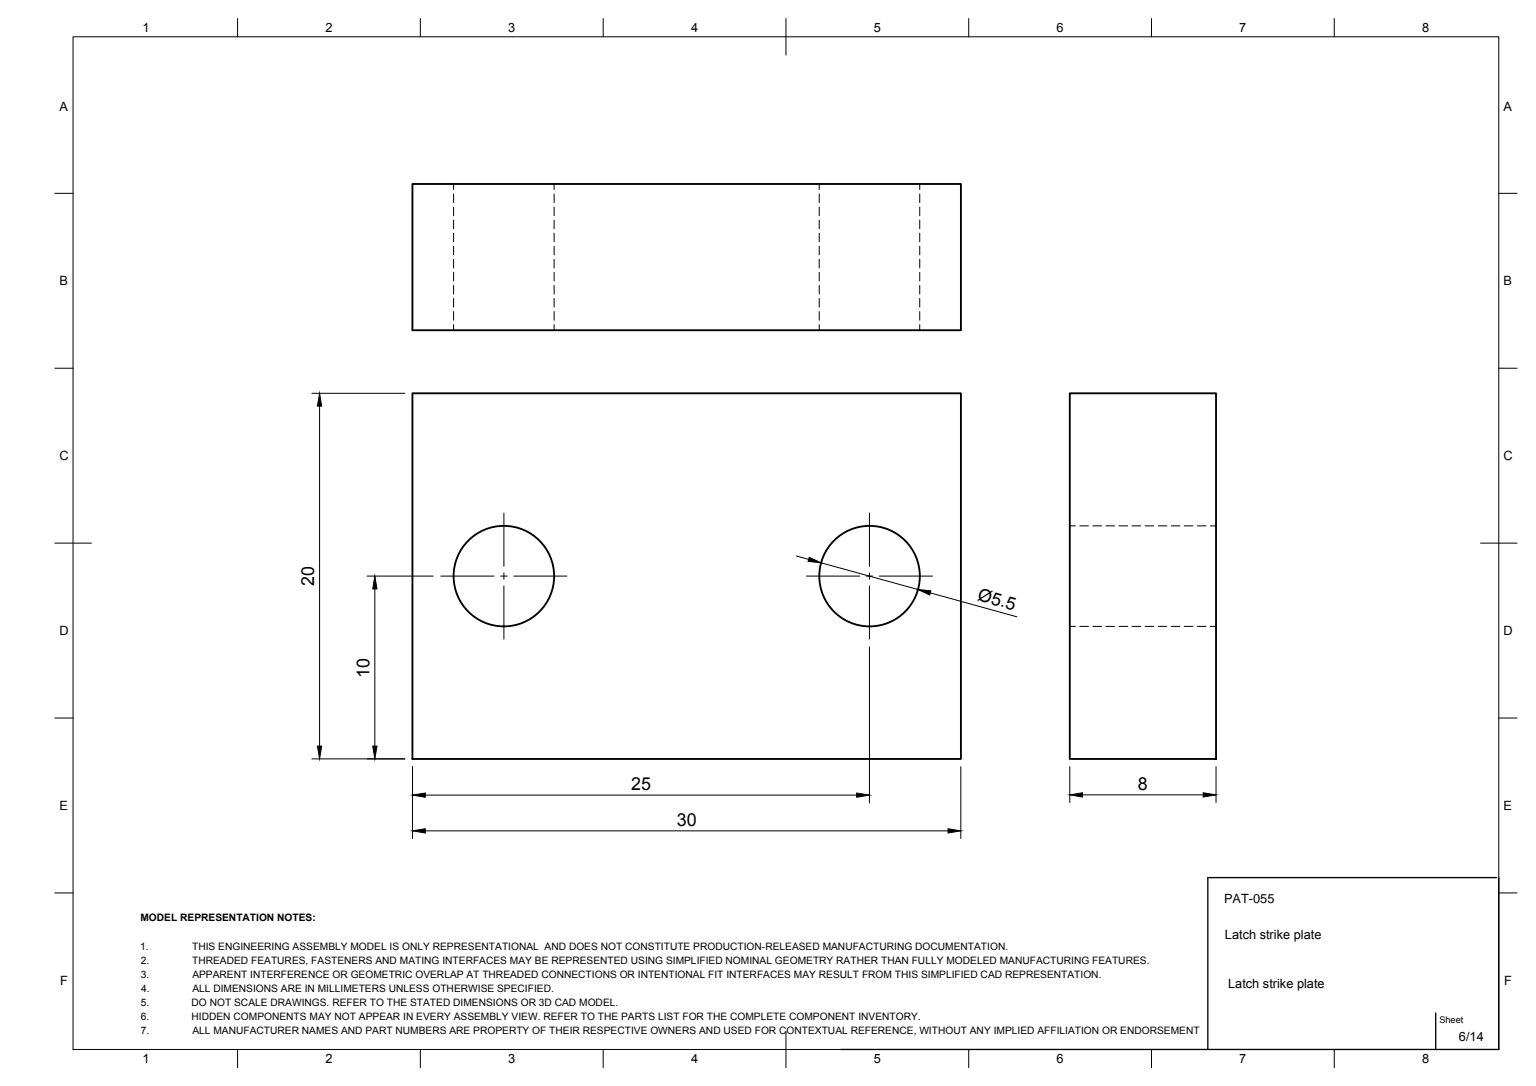
ISO-10303-21;
HEADER;
/* Generated by software containing ST-Developer
 * from STEP Tools, Inc. (www.steptools.com) 
 */

FILE_DESCRIPTION(
/* description */ ('Hinged panel with latch'),
/* implementation_level */ '2;1');

FILE_NAME(
/* name */ 'Latch strike plate.step',
/* time_stamp */ '2026-10-27T20:36:01-07:00',
/* author */ (''),
/* organization */ (''),
/* preprocessor_version */ 'ST-DEVELOPER v20.2',
/* originating_system */ 'Autodesk Translation Framework v15.17.0.0',
/* authorisation */ '');

FILE_SCHEMA (('AUTOMOTIVE_DESIGN { 1 0 10303 214 3 1 1 }'));
ENDSEC;

DATA;
#10=MECHANICAL_DESIGN_GEOMETRIC_PRESENTATION_REPRESENTATION('',(#296),#6743);
#264=SHAPE_REPRESENTATION_RELATIONSHIP('SRR','None',#6839,#280);
#280=ADVANCED_BREP_SHAPE_REPRESENTATION('',(#312),#6725);
#296=STYLED_ITEM('',(#6989),#312);
#312=MANIFOLD_SOLID_BREP('Body1',#3798);
#325=FACE_BOUND('',#732,.T.);
#326=FACE_BOUND('',#733,.T.);
#327=FACE_BOUND('',#736,.T.);
#328=FACE_BOUND('',#737,.T.);
#372=PLANE('',#4003);
#373=PLANE('',#4004);
#374=PLANE('',#4005);
#375=PLANE('',#4006);
#376=PLANE('',#4007);
#377=PLANE('',#4008);
#523=FACE_OUTER_BOUND('',#729,.T.);
#524=FACE_OUTER_BOUND('',#730,.T.);
#525=FACE_OUTER_BOUND('',#731,.T.);
#526=FACE_OUTER_BOUND('',#734,.T.);
#527=FACE_OUTER_BOUND('',#735,.T.);
#528=FACE_OUTER_BOUND('',#738,.T.);
#529=FACE_OUTER_BOUND('',#739,.T.);
#530=FACE_OUTER_BOUND('',#740,.T.);
#729=EDGE_LOOP('',(#2590,#2591,#2592,#2593));
#730=EDGE_LOOP('',(#2594,#2595,#2596,#2597));
#731=EDGE_LOOP('',(#2598,#2599,#2600,#2601));
#732=EDGE_LOOP('',(#2602));
#733=EDGE_LOOP('',(#2603));
#734=EDGE_LOOP('',(#2604,#2605,#2606,#2607));
#735=EDGE_LOOP('',(#2608,#2609,#2610,#2611));
#736=EDGE_LOOP('',(#2612));
#737=EDGE_LOOP('',(#2613));
#738=EDGE_LOOP('',(#2614,#2615,#2616,#2617));
#739=EDGE_LOOP('',(#2618,#2619,#2620,#2621));
#740=EDGE_LOOP('',(#2622,#2623,#2624,#2625));
#982=LINE('',#5469,#1340);
#983=LINE('',#5475,#1341);
#984=LINE('',#5480,#1342);
#985=LINE('',#5482,#1343);
#986=LINE('',#5484,#1344);
#987=LINE('',#5485,#1345);
#988=LINE('',#5488,#1346);
#989=LINE('',#5490,#1347);
#990=LINE('',#5491,#1348);
#991=LINE('',#5494,#1349);
#992=LINE('',#5496,#1350);
#993=LINE('',#5497,#1351);
#994=LINE('',#5499,#1352);
#995=LINE('',#5500,#1353);
#1340=VECTOR('',#4374,0.274999999999999);
#1341=VECTOR('',#4381,0.274999999999999);
#1342=VECTOR('',#4386,1.);
#1343=VECTOR('',#4387,1.);
#1344=VECTOR('',#4388,1.);
#1345=VECTOR('',#4389,1.);
#1346=VECTOR('',#4392,1.);
#1347=VECTOR('',#4393,1.);
#1348=VECTOR('',#4394,1.);
#1349=VECTOR('',#4397,1.);
#1350=VECTOR('',#4398,1.);
#1351=VECTOR('',#4399,1.);
#1352=VECTOR('',#4402,1.);
#1353=VECTOR('',#4403,1.);
#1698=CIRCLE('',#3998,0.274999999999999);
#1699=CIRCLE('',#3999,0.274999999999999);
#1700=CIRCLE('',#4001,0.274999999999999);
#1701=CIRCLE('',#4002,0.274999999999999);
#1791=VERTEX_POINT('',#5466);
#1792=VERTEX_POINT('',#5468);
#1793=VERTEX_POINT('',#5472);
#1794=VERTEX_POINT('',#5474);
#1795=VERTEX_POINT('',#5478);
#1796=VERTEX_POINT('',#5479);
#1797=VERTEX_POINT('',#5481);
#1798=VERTEX_POINT('',#5483);
#1799=VERTEX_POINT('',#5487);
#1800=VERTEX_POINT('',#5489);
#1801=VERTEX_POINT('',#5493);
#1802=VERTEX_POINT('',#5495);
#2107=EDGE_CURVE('',#1791,#1791,#1698,.T.);
#2108=EDGE_CURVE('',#1791,#1792,#982,.T.);
#2109=EDGE_CURVE('',#1792,#1792,#1699,.T.);
#2110=EDGE_CURVE('',#1793,#1793,#1700,.T.);
#2111=EDGE_CURVE('',#1793,#1794,#983,.T.);
#2112=EDGE_CURVE('',#1794,#1794,#1701,.T.);
#2113=EDGE_CURVE('',#1795,#1796,#984,.T.);
#2114=EDGE_CURVE('',#1796,#1797,#985,.T.);
#2115=EDGE_CURVE('',#1798,#1797,#986,.T.);
#2116=EDGE_CURVE('',#1795,#1798,#987,.T.);
#2117=EDGE_CURVE('',#1799,#1795,#988,.T.);
#2118=EDGE_CURVE('',#1800,#1798,#989,.T.);
#2119=EDGE_CURVE('',#1799,#1800,#990,.T.);
#2120=EDGE_CURVE('',#1801,#1799,#991,.T.);
#2121=EDGE_CURVE('',#1802,#1800,#992,.T.);
#2122=EDGE_CURVE('',#1801,#1802,#993,.T.);
#2123=EDGE_CURVE('',#1796,#1801,#994,.T.);
#2124=EDGE_CURVE('',#1797,#1802,#995,.T.);
#2590=ORIENTED_EDGE('',*,*,#2107,.F.);
#2591=ORIENTED_EDGE('',*,*,#2108,.T.);
#2592=ORIENTED_EDGE('',*,*,#2109,.F.);
#2593=ORIENTED_EDGE('',*,*,#2108,.F.);
#2594=ORIENTED_EDGE('',*,*,#2110,.F.);
#2595=ORIENTED_EDGE('',*,*,#2111,.T.);
#2596=ORIENTED_EDGE('',*,*,#2112,.F.);
#2597=ORIENTED_EDGE('',*,*,#2111,.F.);
#2598=ORIENTED_EDGE('',*,*,#2113,.T.);
#2599=ORIENTED_EDGE('',*,*,#2114,.T.);
#2600=ORIENTED_EDGE('',*,*,#2115,.F.);
#2601=ORIENTED_EDGE('',*,*,#2116,.F.);
#2602=ORIENTED_EDGE('',*,*,#2109,.T.);
#2603=ORIENTED_EDGE('',*,*,#2112,.T.);
#2604=ORIENTED_EDGE('',*,*,#2117,.T.);
#2605=ORIENTED_EDGE('',*,*,#2116,.T.);
#2606=ORIENTED_EDGE('',*,*,#2118,.F.);
#2607=ORIENTED_EDGE('',*,*,#2119,.F.);
#2608=ORIENTED_EDGE('',*,*,#2120,.T.);
#2609=ORIENTED_EDGE('',*,*,#2119,.T.);
#2610=ORIENTED_EDGE('',*,*,#2121,.F.);
#2611=ORIENTED_EDGE('',*,*,#2122,.F.);
#2612=ORIENTED_EDGE('',*,*,#2107,.T.);
#2613=ORIENTED_EDGE('',*,*,#2110,.T.);
#2614=ORIENTED_EDGE('',*,*,#2123,.T.);
#2615=ORIENTED_EDGE('',*,*,#2122,.T.);
#2616=ORIENTED_EDGE('',*,*,#2124,.F.);
#2617=ORIENTED_EDGE('',*,*,#2114,.F.);
#2618=ORIENTED_EDGE('',*,*,#2124,.T.);
#2619=ORIENTED_EDGE('',*,*,#2121,.T.);
#2620=ORIENTED_EDGE('',*,*,#2118,.T.);
#2621=ORIENTED_EDGE('',*,*,#2115,.T.);
#2622=ORIENTED_EDGE('',*,*,#2123,.F.);
#2623=ORIENTED_EDGE('',*,*,#2113,.F.);
#2624=ORIENTED_EDGE('',*,*,#2117,.F.);
#2625=ORIENTED_EDGE('',*,*,#2120,.F.);
#3556=CYLINDRICAL_SURFACE('',#3997,0.274999999999999);
#3557=CYLINDRICAL_SURFACE('',#4000,0.274999999999999);
#3592=ADVANCED_FACE('',(#523),#3556,.F.);
#3593=ADVANCED_FACE('',(#524),#3557,.F.);
#3594=ADVANCED_FACE('',(#525,#325,#326),#372,.T.);
#3595=ADVANCED_FACE('',(#526),#373,.T.);
#3596=ADVANCED_FACE('',(#527,#327,#328),#374,.T.);
#3597=ADVANCED_FACE('',(#528),#375,.T.);
#3598=ADVANCED_FACE('',(#529),#376,.T.);
#3599=ADVANCED_FACE('',(#530),#377,.F.);
#3798=CLOSED_SHELL('',(#3592,#3593,#3594,#3595,#3596,#3597,#3598,#3599));
#3996=AXIS2_PLACEMENT_3D('',#5464,#4368,#4369);
#3997=AXIS2_PLACEMENT_3D('',#5465,#4370,#4371);
#3998=AXIS2_PLACEMENT_3D('',#5467,#4372,#4373);
#3999=AXIS2_PLACEMENT_3D('',#5470,#4375,#4376);
#4000=AXIS2_PLACEMENT_3D('',#5471,#4377,#4378);
#4001=AXIS2_PLACEMENT_3D('',#5473,#4379,#4380);
#4002=AXIS2_PLACEMENT_3D('',#5476,#4382,#4383);
#4003=AXIS2_PLACEMENT_3D('',#5477,#4384,#4385);
#4004=AXIS2_PLACEMENT_3D('',#5486,#4390,#4391);
#4005=AXIS2_PLACEMENT_3D('',#5492,#4395,#4396);
#4006=AXIS2_PLACEMENT_3D('',#5498,#4400,#4401);
#4007=AXIS2_PLACEMENT_3D('',#5501,#4404,#4405);
#4008=AXIS2_PLACEMENT_3D('',#5502,#4406,#4407);
#4368=DIRECTION('axis',(0.,0.,1.));
#4369=DIRECTION('refdir',(1.,0.,0.));
#4370=DIRECTION('center_axis',(0.,1.,0.));
#4371=DIRECTION('ref_axis',(1.,0.,0.));
#4372=DIRECTION('center_axis',(0.,1.,0.));
#4373=DIRECTION('ref_axis',(1.,0.,0.));
#4374=DIRECTION('',(0.,1.,0.));
#4375=DIRECTION('center_axis',(0.,-1.,0.));
#4376=DIRECTION('ref_axis',(1.,0.,0.));
#4377=DIRECTION('center_axis',(0.,1.,0.));
#4378=DIRECTION('ref_axis',(1.,0.,0.));
#4379=DIRECTION('center_axis',(0.,1.,0.));
#4380=DIRECTION('ref_axis',(1.,0.,0.));
#4381=DIRECTION('',(0.,1.,0.));
#4382=DIRECTION('center_axis',(0.,-1.,0.));
#4383=DIRECTION('ref_axis',(1.,0.,0.));
#4384=DIRECTION('center_axis',(0.,1.,0.));
#4385=DIRECTION('ref_axis',(-1.,0.,0.));
#4386=DIRECTION('',(-1.,0.,0.));
#4387=DIRECTION('',(0.,0.,1.));
#4388=DIRECTION('',(-1.,0.,0.));
#4389=DIRECTION('',(0.,0.,1.));
#4390=DIRECTION('center_axis',(1.,0.,0.));
#4391=DIRECTION('ref_axis',(0.,1.,0.));
#4392=DIRECTION('',(0.,1.,0.));
#4393=DIRECTION('',(0.,1.,0.));
#4394=DIRECTION('',(0.,0.,1.));
#4395=DIRECTION('center_axis',(0.,-1.,0.));
#4396=DIRECTION('ref_axis',(1.,0.,0.));
#4397=DIRECTION('',(1.,0.,0.));
#4398=DIRECTION('',(1.,0.,0.));
#4399=DIRECTION('',(0.,0.,1.));
#4400=DIRECTION('center_axis',(-1.,0.,0.));
#4401=DIRECTION('ref_axis',(0.,-1.,0.));
#4402=DIRECTION('',(0.,-1.,0.));
#4403=DIRECTION('',(0.,-1.,0.));
#4404=DIRECTION('center_axis',(0.,0.,1.));
#4405=DIRECTION('ref_axis',(1.,0.,0.));
#4406=DIRECTION('center_axis',(0.,0.,1.));
#4407=DIRECTION('ref_axis',(1.,0.,0.));
#5464=CARTESIAN_POINT('',(0.,0.,0.));
#5465=CARTESIAN_POINT('Origin',(22.,-1.9,15.));
#5466=CARTESIAN_POINT('',(21.725,-1.8,15.));
#5467=CARTESIAN_POINT('Origin',(22.,-1.8,15.));
#5468=CARTESIAN_POINT('',(21.725,-1.,15.));
#5469=CARTESIAN_POINT('',(21.725,-1.9,15.));
#5470=CARTESIAN_POINT('Origin',(22.,-1.,15.));
#5471=CARTESIAN_POINT('Origin',(22.,-1.9,17.));
#5472=CARTESIAN_POINT('',(21.725,-1.8,17.));
#5473=CARTESIAN_POINT('Origin',(22.,-1.8,17.));
#5474=CARTESIAN_POINT('',(21.725,-1.,17.));
#5475=CARTESIAN_POINT('',(21.725,-1.9,17.));
#5476=CARTESIAN_POINT('Origin',(22.,-1.,17.));
#5477=CARTESIAN_POINT('Origin',(23.,-1.,14.5));
#5478=CARTESIAN_POINT('',(23.,-1.,14.5));
#5479=CARTESIAN_POINT('',(21.,-1.,14.5));
#5480=CARTESIAN_POINT('',(23.,-1.,14.5));
#5481=CARTESIAN_POINT('',(21.,-1.,17.5));
#5482=CARTESIAN_POINT('',(21.,-1.,14.5));
#5483=CARTESIAN_POINT('',(23.,-1.,17.5));
#5484=CARTESIAN_POINT('',(23.,-1.,17.5));
#5485=CARTESIAN_POINT('',(23.,-1.,14.5));
#5486=CARTESIAN_POINT('Origin',(23.,-1.8,14.5));
#5487=CARTESIAN_POINT('',(23.,-1.8,14.5));
#5488=CARTESIAN_POINT('',(23.,-1.8,14.5));
#5489=CARTESIAN_POINT('',(23.,-1.8,17.5));
#5490=CARTESIAN_POINT('',(23.,-1.8,17.5));
#5491=CARTESIAN_POINT('',(23.,-1.8,14.5));
#5492=CARTESIAN_POINT('Origin',(21.,-1.8,14.5));
#5493=CARTESIAN_POINT('',(21.,-1.8,14.5));
#5494=CARTESIAN_POINT('',(21.,-1.8,14.5));
#5495=CARTESIAN_POINT('',(21.,-1.8,17.5));
#5496=CARTESIAN_POINT('',(21.,-1.8,17.5));
#5497=CARTESIAN_POINT('',(21.,-1.8,14.5));
#5498=CARTESIAN_POINT('Origin',(21.,-1.,14.5));
#5499=CARTESIAN_POINT('',(21.,-1.,14.5));
#5500=CARTESIAN_POINT('',(21.,-1.,17.5));
#5501=CARTESIAN_POINT('Origin',(22.,-1.4,17.5));
#5502=CARTESIAN_POINT('Origin',(22.,-1.4,14.5));
#6704=UNCERTAINTY_MEASURE_WITH_UNIT(LENGTH_MEASURE(0.001),#6744,
'DISTANCE_ACCURACY_VALUE',
'Maximum model space distance between geometric entities at asserted c
onnectivities');
#6722=UNCERTAINTY_MEASURE_WITH_UNIT(LENGTH_MEASURE(0.001),#6744,
'DISTANCE_ACCURACY_VALUE',
'Maximum model space distance between geometric entities at asserted c
onnectivities');
#6725=(
GEOMETRIC_REPRESENTATION_CONTEXT(3)
GLOBAL_UNCERTAINTY_ASSIGNED_CONTEXT((#6704))
GLOBAL_UNIT_ASSIGNED_CONTEXT((#6744,#6746,#6747))
REPRESENTATION_CONTEXT('','3D')
);
#6743=(
GEOMETRIC_REPRESENTATION_CONTEXT(3)
GLOBAL_UNCERTAINTY_ASSIGNED_CONTEXT((#6722))
GLOBAL_UNIT_ASSIGNED_CONTEXT((#6744,#6746,#6747))
REPRESENTATION_CONTEXT('','3D')
);
#6744=(
LENGTH_UNIT()
NAMED_UNIT(*)
SI_UNIT(.CENTI.,.METRE.)
);
#6746=(
NAMED_UNIT(*)
PLANE_ANGLE_UNIT()
SI_UNIT($,.RADIAN.)
);
#6747=(
NAMED_UNIT(*)
SI_UNIT($,.STERADIAN.)
SOLID_ANGLE_UNIT()
);
#6750=SHAPE_DEFINITION_REPRESENTATION(#6770,#6839);
#6770=PRODUCT_DEFINITION_SHAPE('',$,#6860);
#6839=SHAPE_REPRESENTATION('',(#3996),#6725);
#6857=PRODUCT_DEFINITION_CONTEXT('part definition',#6919,'design');
#6860=PRODUCT_DEFINITION('Latch strike plate','Latch strike plate',#6880,
#6857);
#6880=PRODUCT_DEFINITION_FORMATION('',$,#6923);
#6919=APPLICATION_CONTEXT(
'Core Data for Automotive Mechanical Design Process');
#6920=PRODUCT_CONTEXT('part definition',#6919,'mechanical');
#6923=PRODUCT('Latch strike plate','Latch strike plate',
'Latch strike plate',(#6920));
#6983=COLOUR_RGB('Light Blue',0.38,0.62,0.78);
#6984=FILL_AREA_STYLE_COLOUR('',#6983);
#6985=FILL_AREA_STYLE('',(#6984));
#6986=SURFACE_STYLE_FILL_AREA(#6985);
#6987=SURFACE_SIDE_STYLE('',(#6986));
#6988=SURFACE_STYLE_USAGE(.BOTH.,#6987);
#6989=PRESENTATION_STYLE_ASSIGNMENT((#6988));
ENDSEC;
END-ISO-10303-21;
